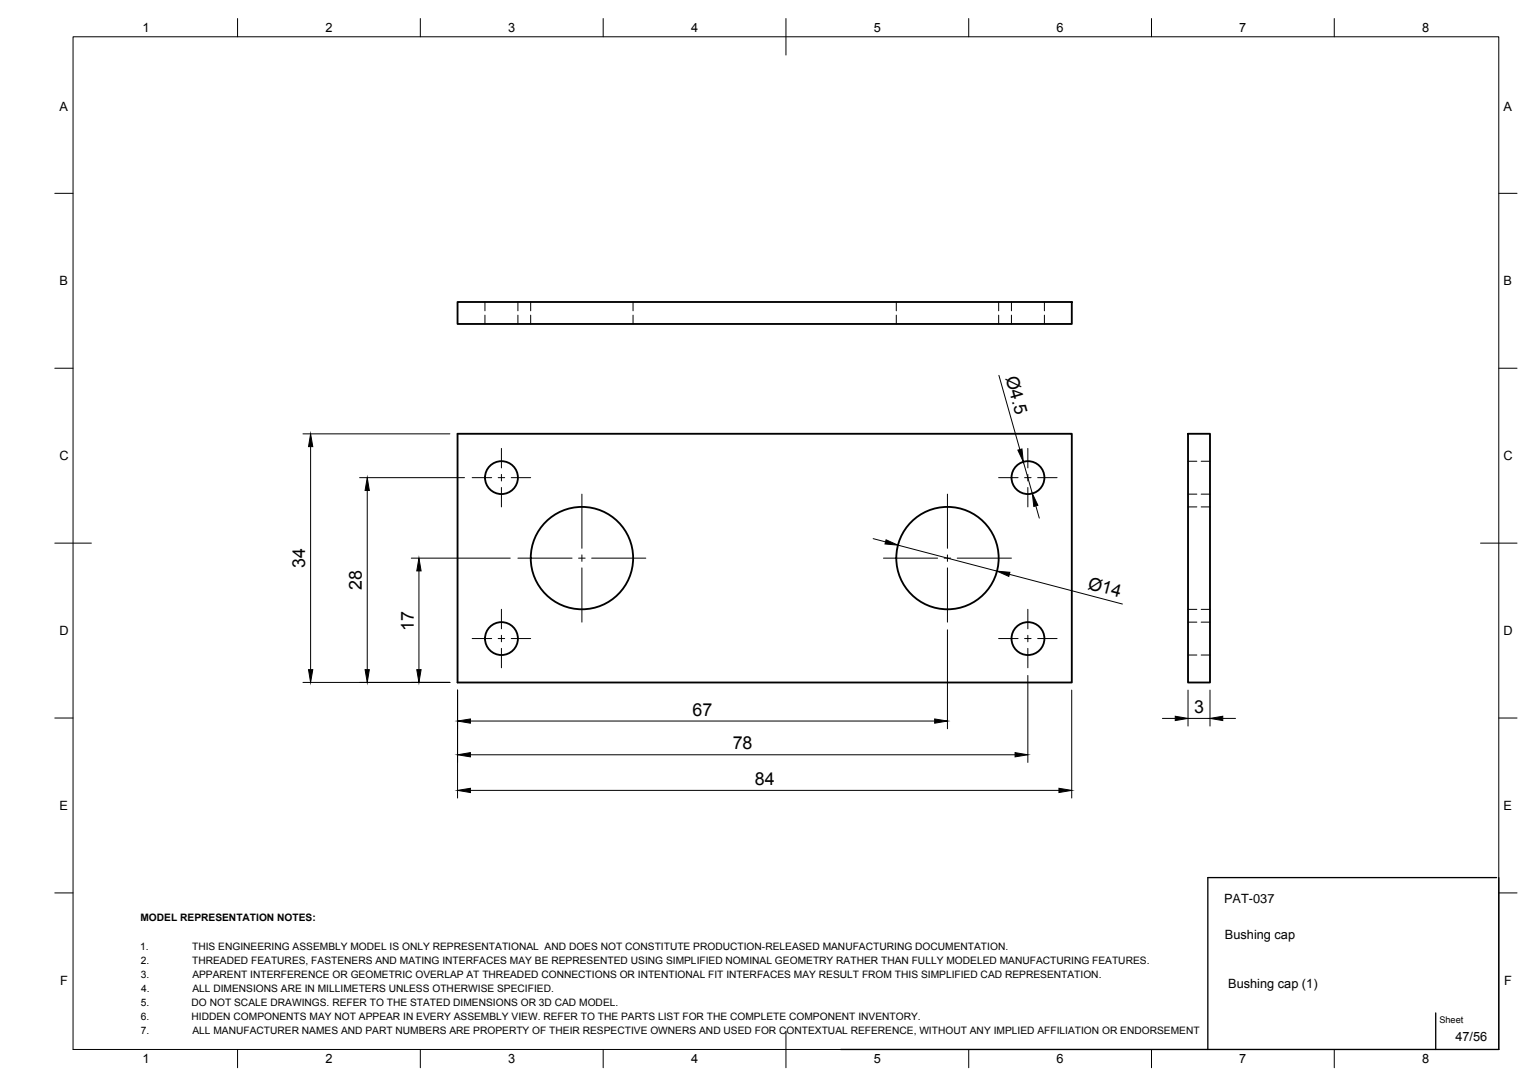
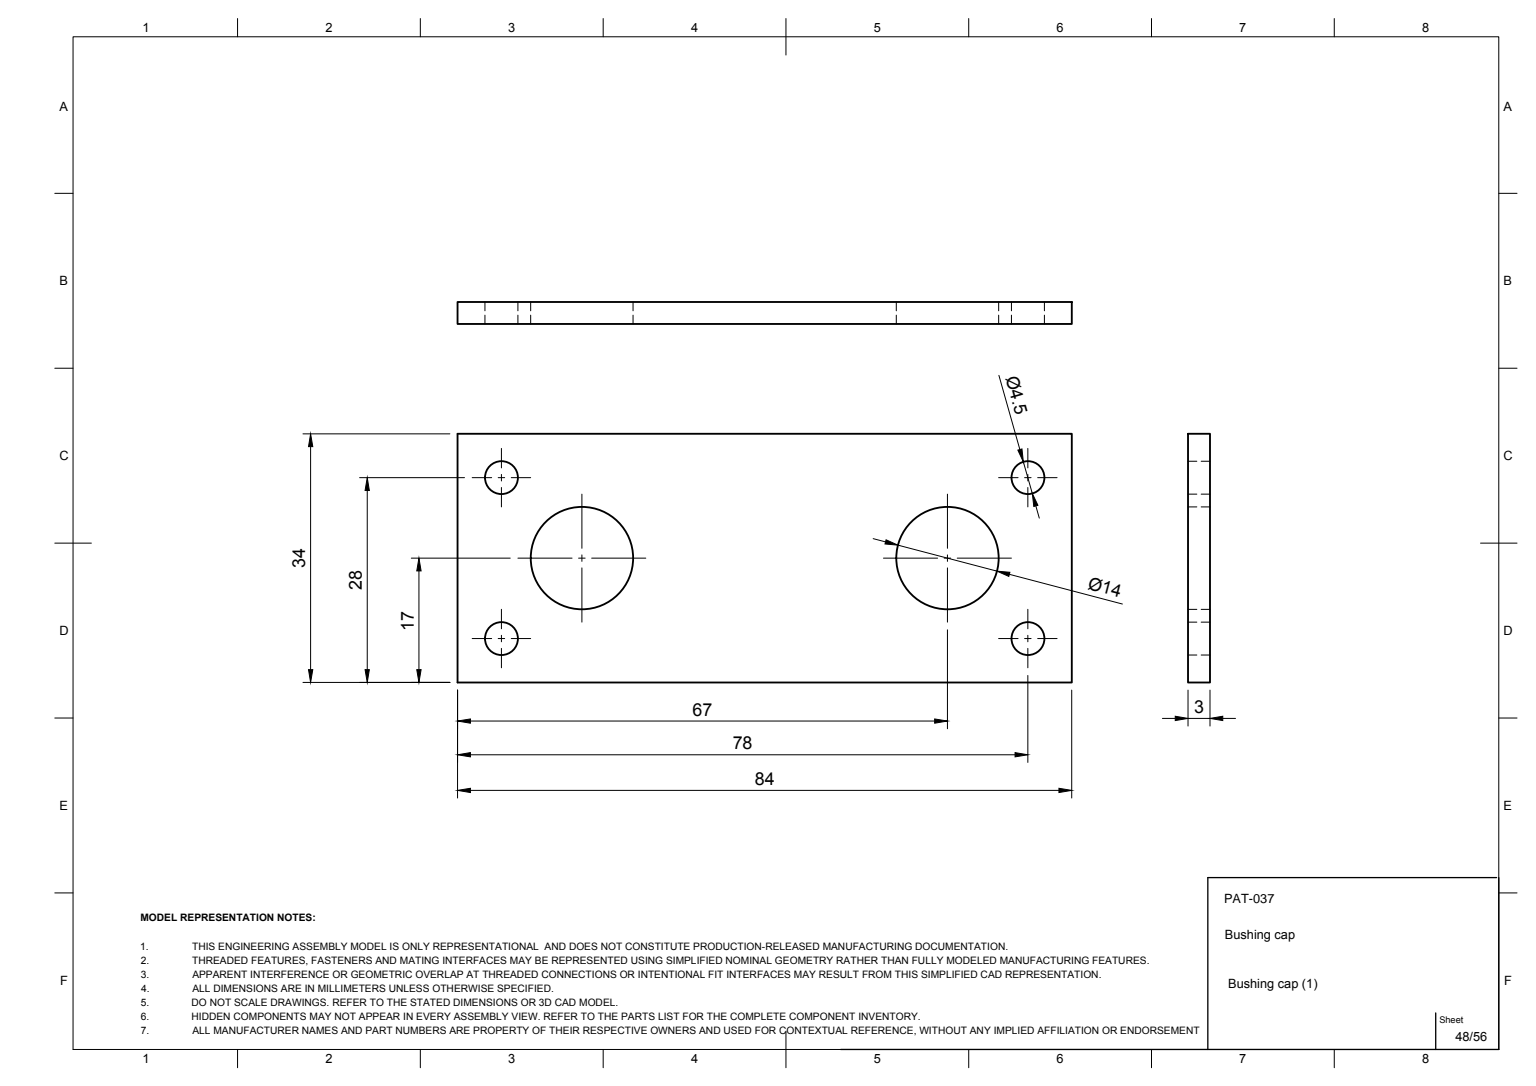
ISO-10303-21;
HEADER;
/* Generated by software containing ST-Developer
 * from STEP Tools, Inc. (www.steptools.com) 
 */

FILE_DESCRIPTION(
/* description */ ('Flywheel Crank-Slider'),
/* implementation_level */ '2;1');

FILE_NAME(
/* name */ 'Bushing cap.step',
/* time_stamp */ '2026-10-28T03:23:13-07:00',
/* author */ (''),
/* organization */ (''),
/* preprocessor_version */ 'ST-DEVELOPER v20.2',
/* originating_system */ 'Autodesk Translation Framework v15.17.0.0',
/* authorisation */ '');

FILE_SCHEMA (('AUTOMOTIVE_DESIGN { 1 0 10303 214 3 1 1 }'));
ENDSEC;

DATA;
#10=MECHANICAL_DESIGN_GEOMETRIC_PRESENTATION_REPRESENTATION('',(#720),#17322);
#607=SHAPE_REPRESENTATION_RELATIONSHIP('SRR','None',#17608,#659);
#659=ADVANCED_BREP_SHAPE_REPRESENTATION('',(#777),#17312);
#720=STYLED_ITEM('',(#17924),#777);
#777=MANIFOLD_SOLID_BREP('Body1',#9102);
#967=FACE_BOUND('',#2496,.T.);
#968=FACE_BOUND('',#2497,.T.);
#969=FACE_BOUND('',#2498,.T.);
#970=FACE_BOUND('',#2499,.T.);
#971=FACE_BOUND('',#2500,.T.);
#972=FACE_BOUND('',#2501,.T.);
#973=FACE_BOUND('',#2504,.T.);
#974=FACE_BOUND('',#2505,.T.);
#975=FACE_BOUND('',#2506,.T.);
#976=FACE_BOUND('',#2507,.T.);
#977=FACE_BOUND('',#2508,.T.);
#978=FACE_BOUND('',#2509,.T.);
#1270=PLANE('',#10587);
#1271=PLANE('',#10588);
#1272=PLANE('',#10589);
#1273=PLANE('',#10590);
#1274=PLANE('',#10591);
#1275=PLANE('',#10592);
#1771=FACE_OUTER_BOUND('',#2488,.T.);
#1772=FACE_OUTER_BOUND('',#2489,.T.);
#1773=FACE_OUTER_BOUND('',#2490,.T.);
#1774=FACE_OUTER_BOUND('',#2491,.T.);
#1775=FACE_OUTER_BOUND('',#2492,.T.);
#1776=FACE_OUTER_BOUND('',#2493,.T.);
#1777=FACE_OUTER_BOUND('',#2494,.T.);
#1778=FACE_OUTER_BOUND('',#2495,.T.);
#1779=FACE_OUTER_BOUND('',#2502,.T.);
#1780=FACE_OUTER_BOUND('',#2503,.T.);
#1781=FACE_OUTER_BOUND('',#2510,.T.);
#1782=FACE_OUTER_BOUND('',#2511,.T.);
#2488=EDGE_LOOP('',(#8000,#8001,#8002,#8003));
#2489=EDGE_LOOP('',(#8004,#8005,#8006,#8007));
#2490=EDGE_LOOP('',(#8008,#8009,#8010,#8011));
#2491=EDGE_LOOP('',(#8012,#8013,#8014,#8015));
#2492=EDGE_LOOP('',(#8016,#8017,#8018,#8019));
#2493=EDGE_LOOP('',(#8020,#8021,#8022,#8023));
#2494=EDGE_LOOP('',(#8024,#8025,#8026,#8027));
#2495=EDGE_LOOP('',(#8028,#8029,#8030,#8031));
#2496=EDGE_LOOP('',(#8032));
#2497=EDGE_LOOP('',(#8033));
#2498=EDGE_LOOP('',(#8034));
#2499=EDGE_LOOP('',(#8035));
#2500=EDGE_LOOP('',(#8036));
#2501=EDGE_LOOP('',(#8037));
#2502=EDGE_LOOP('',(#8038,#8039,#8040,#8041));
#2503=EDGE_LOOP('',(#8042,#8043,#8044,#8045));
#2504=EDGE_LOOP('',(#8046));
#2505=EDGE_LOOP('',(#8047));
#2506=EDGE_LOOP('',(#8048));
#2507=EDGE_LOOP('',(#8049));
#2508=EDGE_LOOP('',(#8050));
#2509=EDGE_LOOP('',(#8051));
#2510=EDGE_LOOP('',(#8052,#8053,#8054,#8055));
#2511=EDGE_LOOP('',(#8056,#8057,#8058,#8059));
#3133=LINE('',#16741,#3744);
#3134=LINE('',#16747,#3745);
#3135=LINE('',#16753,#3746);
#3136=LINE('',#16759,#3747);
#3137=LINE('',#16765,#3748);
#3138=LINE('',#16771,#3749);
#3139=LINE('',#16776,#3750);
#3140=LINE('',#16778,#3751);
#3141=LINE('',#16780,#3752);
#3142=LINE('',#16781,#3753);
#3143=LINE('',#16784,#3754);
#3144=LINE('',#16786,#3755);
#3145=LINE('',#16787,#3756);
#3146=LINE('',#16790,#3757);
#3147=LINE('',#16792,#3758);
#3148=LINE('',#16793,#3759);
#3149=LINE('',#16795,#3760);
#3150=LINE('',#16796,#3761);
#3744=VECTOR('',#13119,0.225);
#3745=VECTOR('',#13126,0.225);
#3746=VECTOR('',#13133,0.225);
#3747=VECTOR('',#13140,0.225);
#3748=VECTOR('',#13147,0.7);
#3749=VECTOR('',#13154,0.7);
#3750=VECTOR('',#13159,1.);
#3751=VECTOR('',#13160,1.);
#3752=VECTOR('',#13161,1.);
#3753=VECTOR('',#13162,1.);
#3754=VECTOR('',#13165,1.);
#3755=VECTOR('',#13166,1.);
#3756=VECTOR('',#13167,1.);
#3757=VECTOR('',#13170,1.);
#3758=VECTOR('',#13171,1.);
#3759=VECTOR('',#13172,1.);
#3760=VECTOR('',#13175,1.);
#3761=VECTOR('',#13176,1.);
#4206=CIRCLE('',#10570,0.225);
#4207=CIRCLE('',#10571,0.225);
#4208=CIRCLE('',#10573,0.225);
#4209=CIRCLE('',#10574,0.225);
#4210=CIRCLE('',#10576,0.225);
#4211=CIRCLE('',#10577,0.225);
#4212=CIRCLE('',#10579,0.225);
#4213=CIRCLE('',#10580,0.225);
#4214=CIRCLE('',#10582,0.7);
#4215=CIRCLE('',#10583,0.7);
#4216=CIRCLE('',#10585,0.7);
#4217=CIRCLE('',#10586,0.7);
#4909=VERTEX_POINT('',#16738);
#4910=VERTEX_POINT('',#16740);
#4911=VERTEX_POINT('',#16744);
#4912=VERTEX_POINT('',#16746);
#4913=VERTEX_POINT('',#16750);
#4914=VERTEX_POINT('',#16752);
#4915=VERTEX_POINT('',#16756);
#4916=VERTEX_POINT('',#16758);
#4917=VERTEX_POINT('',#16762);
#4918=VERTEX_POINT('',#16764);
#4919=VERTEX_POINT('',#16768);
#4920=VERTEX_POINT('',#16770);
#4921=VERTEX_POINT('',#16774);
#4922=VERTEX_POINT('',#16775);
#4923=VERTEX_POINT('',#16777);
#4924=VERTEX_POINT('',#16779);
#4925=VERTEX_POINT('',#16783);
#4926=VERTEX_POINT('',#16785);
#4927=VERTEX_POINT('',#16789);
#4928=VERTEX_POINT('',#16791);
#5957=EDGE_CURVE('',#4909,#4909,#4206,.T.);
#5958=EDGE_CURVE('',#4909,#4910,#3133,.T.);
#5959=EDGE_CURVE('',#4910,#4910,#4207,.T.);
#5960=EDGE_CURVE('',#4911,#4911,#4208,.T.);
#5961=EDGE_CURVE('',#4911,#4912,#3134,.T.);
#5962=EDGE_CURVE('',#4912,#4912,#4209,.T.);
#5963=EDGE_CURVE('',#4913,#4913,#4210,.T.);
#5964=EDGE_CURVE('',#4913,#4914,#3135,.T.);
#5965=EDGE_CURVE('',#4914,#4914,#4211,.T.);
#5966=EDGE_CURVE('',#4915,#4915,#4212,.T.);
#5967=EDGE_CURVE('',#4915,#4916,#3136,.T.);
#5968=EDGE_CURVE('',#4916,#4916,#4213,.T.);
#5969=EDGE_CURVE('',#4917,#4917,#4214,.T.);
#5970=EDGE_CURVE('',#4917,#4918,#3137,.T.);
#5971=EDGE_CURVE('',#4918,#4918,#4215,.T.);
#5972=EDGE_CURVE('',#4919,#4919,#4216,.T.);
#5973=EDGE_CURVE('',#4919,#4920,#3138,.T.);
#5974=EDGE_CURVE('',#4920,#4920,#4217,.T.);
#5975=EDGE_CURVE('',#4921,#4922,#3139,.T.);
#5976=EDGE_CURVE('',#4922,#4923,#3140,.T.);
#5977=EDGE_CURVE('',#4924,#4923,#3141,.T.);
#5978=EDGE_CURVE('',#4921,#4924,#3142,.T.);
#5979=EDGE_CURVE('',#4925,#4921,#3143,.T.);
#5980=EDGE_CURVE('',#4926,#4924,#3144,.T.);
#5981=EDGE_CURVE('',#4925,#4926,#3145,.T.);
#5982=EDGE_CURVE('',#4927,#4925,#3146,.T.);
#5983=EDGE_CURVE('',#4928,#4926,#3147,.T.);
#5984=EDGE_CURVE('',#4927,#4928,#3148,.T.);
#5985=EDGE_CURVE('',#4922,#4927,#3149,.T.);
#5986=EDGE_CURVE('',#4923,#4928,#3150,.T.);
#8000=ORIENTED_EDGE('',*,*,#5957,.F.);
#8001=ORIENTED_EDGE('',*,*,#5958,.T.);
#8002=ORIENTED_EDGE('',*,*,#5959,.F.);
#8003=ORIENTED_EDGE('',*,*,#5958,.F.);
#8004=ORIENTED_EDGE('',*,*,#5960,.F.);
#8005=ORIENTED_EDGE('',*,*,#5961,.T.);
#8006=ORIENTED_EDGE('',*,*,#5962,.F.);
#8007=ORIENTED_EDGE('',*,*,#5961,.F.);
#8008=ORIENTED_EDGE('',*,*,#5963,.F.);
#8009=ORIENTED_EDGE('',*,*,#5964,.T.);
#8010=ORIENTED_EDGE('',*,*,#5965,.F.);
#8011=ORIENTED_EDGE('',*,*,#5964,.F.);
#8012=ORIENTED_EDGE('',*,*,#5966,.F.);
#8013=ORIENTED_EDGE('',*,*,#5967,.T.);
#8014=ORIENTED_EDGE('',*,*,#5968,.F.);
#8015=ORIENTED_EDGE('',*,*,#5967,.F.);
#8016=ORIENTED_EDGE('',*,*,#5969,.F.);
#8017=ORIENTED_EDGE('',*,*,#5970,.T.);
#8018=ORIENTED_EDGE('',*,*,#5971,.F.);
#8019=ORIENTED_EDGE('',*,*,#5970,.F.);
#8020=ORIENTED_EDGE('',*,*,#5972,.F.);
#8021=ORIENTED_EDGE('',*,*,#5973,.T.);
#8022=ORIENTED_EDGE('',*,*,#5974,.F.);
#8023=ORIENTED_EDGE('',*,*,#5973,.F.);
#8024=ORIENTED_EDGE('',*,*,#5975,.T.);
#8025=ORIENTED_EDGE('',*,*,#5976,.T.);
#8026=ORIENTED_EDGE('',*,*,#5977,.F.);
#8027=ORIENTED_EDGE('',*,*,#5978,.F.);
#8028=ORIENTED_EDGE('',*,*,#5979,.T.);
#8029=ORIENTED_EDGE('',*,*,#5978,.T.);
#8030=ORIENTED_EDGE('',*,*,#5980,.F.);
#8031=ORIENTED_EDGE('',*,*,#5981,.F.);
#8032=ORIENTED_EDGE('',*,*,#5974,.T.);
#8033=ORIENTED_EDGE('',*,*,#5971,.T.);
#8034=ORIENTED_EDGE('',*,*,#5968,.T.);
#8035=ORIENTED_EDGE('',*,*,#5965,.T.);
#8036=ORIENTED_EDGE('',*,*,#5962,.T.);
#8037=ORIENTED_EDGE('',*,*,#5959,.T.);
#8038=ORIENTED_EDGE('',*,*,#5982,.T.);
#8039=ORIENTED_EDGE('',*,*,#5981,.T.);
#8040=ORIENTED_EDGE('',*,*,#5983,.F.);
#8041=ORIENTED_EDGE('',*,*,#5984,.F.);
#8042=ORIENTED_EDGE('',*,*,#5985,.T.);
#8043=ORIENTED_EDGE('',*,*,#5984,.T.);
#8044=ORIENTED_EDGE('',*,*,#5986,.F.);
#8045=ORIENTED_EDGE('',*,*,#5976,.F.);
#8046=ORIENTED_EDGE('',*,*,#5972,.T.);
#8047=ORIENTED_EDGE('',*,*,#5969,.T.);
#8048=ORIENTED_EDGE('',*,*,#5966,.T.);
#8049=ORIENTED_EDGE('',*,*,#5963,.T.);
#8050=ORIENTED_EDGE('',*,*,#5960,.T.);
#8051=ORIENTED_EDGE('',*,*,#5957,.T.);
#8052=ORIENTED_EDGE('',*,*,#5986,.T.);
#8053=ORIENTED_EDGE('',*,*,#5983,.T.);
#8054=ORIENTED_EDGE('',*,*,#5980,.T.);
#8055=ORIENTED_EDGE('',*,*,#5977,.T.);
#8056=ORIENTED_EDGE('',*,*,#5985,.F.);
#8057=ORIENTED_EDGE('',*,*,#5975,.F.);
#8058=ORIENTED_EDGE('',*,*,#5979,.F.);
#8059=ORIENTED_EDGE('',*,*,#5982,.F.);
#8480=CYLINDRICAL_SURFACE('',#10569,0.225);
#8481=CYLINDRICAL_SURFACE('',#10572,0.225);
#8482=CYLINDRICAL_SURFACE('',#10575,0.225);
#8483=CYLINDRICAL_SURFACE('',#10578,0.225);
#8484=CYLINDRICAL_SURFACE('',#10581,0.7);
#8485=CYLINDRICAL_SURFACE('',#10584,0.7);
#8962=ADVANCED_FACE('',(#1771),#8480,.F.);
#8963=ADVANCED_FACE('',(#1772),#8481,.F.);
#8964=ADVANCED_FACE('',(#1773),#8482,.F.);
#8965=ADVANCED_FACE('',(#1774),#8483,.F.);
#8966=ADVANCED_FACE('',(#1775),#8484,.F.);
#8967=ADVANCED_FACE('',(#1776),#8485,.F.);
#8968=ADVANCED_FACE('',(#1777),#1270,.T.);
#8969=ADVANCED_FACE('',(#1778,#967,#968,#969,#970,#971,#972),#1271,.T.);
#8970=ADVANCED_FACE('',(#1779),#1272,.T.);
#8971=ADVANCED_FACE('',(#1780,#973,#974,#975,#976,#977,#978),#1273,.T.);
#8972=ADVANCED_FACE('',(#1781),#1274,.T.);
#8973=ADVANCED_FACE('',(#1782),#1275,.F.);
#9102=CLOSED_SHELL('',(#8962,#8963,#8964,#8965,#8966,#8967,#8968,#8969,
#8970,#8971,#8972,#8973));
#10568=AXIS2_PLACEMENT_3D('',#16736,#13113,#13114);
#10569=AXIS2_PLACEMENT_3D('',#16737,#13115,#13116);
#10570=AXIS2_PLACEMENT_3D('',#16739,#13117,#13118);
#10571=AXIS2_PLACEMENT_3D('',#16742,#13120,#13121);
#10572=AXIS2_PLACEMENT_3D('',#16743,#13122,#13123);
#10573=AXIS2_PLACEMENT_3D('',#16745,#13124,#13125);
#10574=AXIS2_PLACEMENT_3D('',#16748,#13127,#13128);
#10575=AXIS2_PLACEMENT_3D('',#16749,#13129,#13130);
#10576=AXIS2_PLACEMENT_3D('',#16751,#13131,#13132);
#10577=AXIS2_PLACEMENT_3D('',#16754,#13134,#13135);
#10578=AXIS2_PLACEMENT_3D('',#16755,#13136,#13137);
#10579=AXIS2_PLACEMENT_3D('',#16757,#13138,#13139);
#10580=AXIS2_PLACEMENT_3D('',#16760,#13141,#13142);
#10581=AXIS2_PLACEMENT_3D('',#16761,#13143,#13144);
#10582=AXIS2_PLACEMENT_3D('',#16763,#13145,#13146);
#10583=AXIS2_PLACEMENT_3D('',#16766,#13148,#13149);
#10584=AXIS2_PLACEMENT_3D('',#16767,#13150,#13151);
#10585=AXIS2_PLACEMENT_3D('',#16769,#13152,#13153);
#10586=AXIS2_PLACEMENT_3D('',#16772,#13155,#13156);
#10587=AXIS2_PLACEMENT_3D('',#16773,#13157,#13158);
#10588=AXIS2_PLACEMENT_3D('',#16782,#13163,#13164);
#10589=AXIS2_PLACEMENT_3D('',#16788,#13168,#13169);
#10590=AXIS2_PLACEMENT_3D('',#16794,#13173,#13174);
#10591=AXIS2_PLACEMENT_3D('',#16797,#13177,#13178);
#10592=AXIS2_PLACEMENT_3D('',#16798,#13179,#13180);
#13113=DIRECTION('axis',(0.,0.,1.));
#13114=DIRECTION('refdir',(1.,0.,0.));
#13115=DIRECTION('center_axis',(1.,0.,0.));
#13116=DIRECTION('ref_axis',(0.,0.,-1.));
#13117=DIRECTION('center_axis',(1.,0.,0.));
#13118=DIRECTION('ref_axis',(0.,0.,-1.));
#13119=DIRECTION('',(1.,0.,0.));
#13120=DIRECTION('center_axis',(-1.,0.,0.));
#13121=DIRECTION('ref_axis',(0.,0.,-1.));
#13122=DIRECTION('center_axis',(1.,0.,0.));
#13123=DIRECTION('ref_axis',(0.,0.,-1.));
#13124=DIRECTION('center_axis',(1.,0.,0.));
#13125=DIRECTION('ref_axis',(0.,0.,-1.));
#13126=DIRECTION('',(1.,0.,0.));
#13127=DIRECTION('center_axis',(-1.,0.,0.));
#13128=DIRECTION('ref_axis',(0.,0.,-1.));
#13129=DIRECTION('center_axis',(1.,0.,0.));
#13130=DIRECTION('ref_axis',(0.,0.,-1.));
#13131=DIRECTION('center_axis',(1.,0.,0.));
#13132=DIRECTION('ref_axis',(0.,0.,-1.));
#13133=DIRECTION('',(1.,0.,0.));
#13134=DIRECTION('center_axis',(-1.,0.,0.));
#13135=DIRECTION('ref_axis',(0.,0.,-1.));
#13136=DIRECTION('center_axis',(1.,0.,0.));
#13137=DIRECTION('ref_axis',(0.,0.,-1.));
#13138=DIRECTION('center_axis',(1.,0.,0.));
#13139=DIRECTION('ref_axis',(0.,0.,-1.));
#13140=DIRECTION('',(1.,0.,0.));
#13141=DIRECTION('center_axis',(-1.,0.,0.));
#13142=DIRECTION('ref_axis',(0.,0.,-1.));
#13143=DIRECTION('center_axis',(1.,0.,0.));
#13144=DIRECTION('ref_axis',(0.,0.,-1.));
#13145=DIRECTION('center_axis',(1.,0.,0.));
#13146=DIRECTION('ref_axis',(0.,0.,-1.));
#13147=DIRECTION('',(1.,0.,0.));
#13148=DIRECTION('center_axis',(-1.,0.,0.));
#13149=DIRECTION('ref_axis',(0.,0.,-1.));
#13150=DIRECTION('center_axis',(1.,0.,0.));
#13151=DIRECTION('ref_axis',(0.,0.,-1.));
#13152=DIRECTION('center_axis',(1.,0.,0.));
#13153=DIRECTION('ref_axis',(0.,0.,-1.));
#13154=DIRECTION('',(1.,0.,0.));
#13155=DIRECTION('center_axis',(-1.,0.,0.));
#13156=DIRECTION('ref_axis',(0.,0.,-1.));
#13157=DIRECTION('center_axis',(0.,1.,0.));
#13158=DIRECTION('ref_axis',(-1.,0.,0.));
#13159=DIRECTION('',(-1.,0.,0.));
#13160=DIRECTION('',(0.,0.,1.));
#13161=DIRECTION('',(-1.,0.,0.));
#13162=DIRECTION('',(0.,0.,1.));
#13163=DIRECTION('center_axis',(1.,0.,0.));
#13164=DIRECTION('ref_axis',(0.,1.,0.));
#13165=DIRECTION('',(0.,1.,0.));
#13166=DIRECTION('',(0.,1.,0.));
#13167=DIRECTION('',(0.,0.,1.));
#13168=DIRECTION('center_axis',(0.,-1.,0.));
#13169=DIRECTION('ref_axis',(1.,0.,0.));
#13170=DIRECTION('',(1.,0.,0.));
#13171=DIRECTION('',(1.,0.,0.));
#13172=DIRECTION('',(0.,0.,1.));
#13173=DIRECTION('center_axis',(-1.,0.,0.));
#13174=DIRECTION('ref_axis',(0.,-1.,0.));
#13175=DIRECTION('',(0.,-1.,0.));
#13176=DIRECTION('',(0.,-1.,0.));
#13177=DIRECTION('center_axis',(0.,0.,1.));
#13178=DIRECTION('ref_axis',(1.,0.,0.));
#13179=DIRECTION('center_axis',(0.,0.,1.));
#13180=DIRECTION('ref_axis',(1.,0.,0.));
#16736=CARTESIAN_POINT('',(0.,0.,0.));
#16737=CARTESIAN_POINT('Origin',(10.,3.6,3.9));
#16738=CARTESIAN_POINT('',(10.1,3.6,4.125));
#16739=CARTESIAN_POINT('Origin',(10.1,3.6,3.9));
#16740=CARTESIAN_POINT('',(10.4,3.6,4.125));
#16741=CARTESIAN_POINT('',(10.,3.6,4.125));
#16742=CARTESIAN_POINT('Origin',(10.4,3.6,3.9));
#16743=CARTESIAN_POINT('Origin',(10.,-3.6,6.1));
#16744=CARTESIAN_POINT('',(10.1,-3.6,6.325));
#16745=CARTESIAN_POINT('Origin',(10.1,-3.6,6.1));
#16746=CARTESIAN_POINT('',(10.4,-3.6,6.325));
#16747=CARTESIAN_POINT('',(10.,-3.6,6.325));
#16748=CARTESIAN_POINT('Origin',(10.4,-3.6,6.1));
#16749=CARTESIAN_POINT('Origin',(10.,-3.6,3.9));
#16750=CARTESIAN_POINT('',(10.1,-3.6,4.125));
#16751=CARTESIAN_POINT('Origin',(10.1,-3.6,3.9));
#16752=CARTESIAN_POINT('',(10.4,-3.6,4.125));
#16753=CARTESIAN_POINT('',(10.,-3.6,4.125));
#16754=CARTESIAN_POINT('Origin',(10.4,-3.6,3.9));
#16755=CARTESIAN_POINT('Origin',(10.,3.6,6.1));
#16756=CARTESIAN_POINT('',(10.1,3.6,6.325));
#16757=CARTESIAN_POINT('Origin',(10.1,3.6,6.1));
#16758=CARTESIAN_POINT('',(10.4,3.6,6.325));
#16759=CARTESIAN_POINT('',(10.,3.6,6.325));
#16760=CARTESIAN_POINT('Origin',(10.4,3.6,6.1));
#16761=CARTESIAN_POINT('Origin',(10.,-2.5,5.));
#16762=CARTESIAN_POINT('',(10.1,-2.5,5.7));
#16763=CARTESIAN_POINT('Origin',(10.1,-2.5,5.));
#16764=CARTESIAN_POINT('',(10.4,-2.5,5.7));
#16765=CARTESIAN_POINT('',(10.,-2.5,5.7));
#16766=CARTESIAN_POINT('Origin',(10.4,-2.5,5.));
#16767=CARTESIAN_POINT('Origin',(10.,2.5,5.));
#16768=CARTESIAN_POINT('',(10.1,2.5,5.7));
#16769=CARTESIAN_POINT('Origin',(10.1,2.5,5.));
#16770=CARTESIAN_POINT('',(10.4,2.5,5.7));
#16771=CARTESIAN_POINT('',(10.,2.5,5.7));
#16772=CARTESIAN_POINT('Origin',(10.4,2.5,5.));
#16773=CARTESIAN_POINT('Origin',(10.4,4.2,3.3));
#16774=CARTESIAN_POINT('',(10.4,4.2,3.3));
#16775=CARTESIAN_POINT('',(10.1,4.2,3.3));
#16776=CARTESIAN_POINT('',(10.4,4.2,3.3));
#16777=CARTESIAN_POINT('',(10.1,4.2,6.7));
#16778=CARTESIAN_POINT('',(10.1,4.2,3.3));
#16779=CARTESIAN_POINT('',(10.4,4.2,6.7));
#16780=CARTESIAN_POINT('',(10.4,4.2,6.7));
#16781=CARTESIAN_POINT('',(10.4,4.2,3.3));
#16782=CARTESIAN_POINT('Origin',(10.4,-4.2,3.3));
#16783=CARTESIAN_POINT('',(10.4,-4.2,3.3));
#16784=CARTESIAN_POINT('',(10.4,-4.2,3.3));
#16785=CARTESIAN_POINT('',(10.4,-4.2,6.7));
#16786=CARTESIAN_POINT('',(10.4,-4.2,6.7));
#16787=CARTESIAN_POINT('',(10.4,-4.2,3.3));
#16788=CARTESIAN_POINT('Origin',(10.1,-4.2,3.3));
#16789=CARTESIAN_POINT('',(10.1,-4.2,3.3));
#16790=CARTESIAN_POINT('',(10.1,-4.2,3.3));
#16791=CARTESIAN_POINT('',(10.1,-4.2,6.7));
#16792=CARTESIAN_POINT('',(10.1,-4.2,6.7));
#16793=CARTESIAN_POINT('',(10.1,-4.2,3.3));
#16794=CARTESIAN_POINT('Origin',(10.1,4.2,3.3));
#16795=CARTESIAN_POINT('',(10.1,4.2,3.3));
#16796=CARTESIAN_POINT('',(10.1,4.2,6.7));
#16797=CARTESIAN_POINT('Origin',(10.25,0.,6.7));
#16798=CARTESIAN_POINT('Origin',(10.25,0.,3.3));
#17251=UNCERTAINTY_MEASURE_WITH_UNIT(LENGTH_MEASURE(0.001),#17323,
'DISTANCE_ACCURACY_VALUE',
'Maximum model space distance between geometric entities at asserted c
onnectivities');
#17261=UNCERTAINTY_MEASURE_WITH_UNIT(LENGTH_MEASURE(0.001),#17323,
'DISTANCE_ACCURACY_VALUE',
'Maximum model space distance between geometric entities at asserted c
onnectivities');
#17312=(
GEOMETRIC_REPRESENTATION_CONTEXT(3)
GLOBAL_UNCERTAINTY_ASSIGNED_CONTEXT((#17251))
GLOBAL_UNIT_ASSIGNED_CONTEXT((#17323,#17325,#17326))
REPRESENTATION_CONTEXT('','3D')
);
#17322=(
GEOMETRIC_REPRESENTATION_CONTEXT(3)
GLOBAL_UNCERTAINTY_ASSIGNED_CONTEXT((#17261))
GLOBAL_UNIT_ASSIGNED_CONTEXT((#17323,#17325,#17326))
REPRESENTATION_CONTEXT('','3D')
);
#17323=(
LENGTH_UNIT()
NAMED_UNIT(*)
SI_UNIT(.CENTI.,.METRE.)
);
#17325=(
NAMED_UNIT(*)
PLANE_ANGLE_UNIT()
SI_UNIT($,.RADIAN.)
);
#17326=(
NAMED_UNIT(*)
SI_UNIT($,.STERADIAN.)
SOLID_ANGLE_UNIT()
);
#17377=SHAPE_DEFINITION_REPRESENTATION(#17451,#17608);
#17451=PRODUCT_DEFINITION_SHAPE('',$,#17669);
#17608=SHAPE_REPRESENTATION('',(#10568),#17312);
#17618=PRODUCT_DEFINITION_CONTEXT('part definition',#17800,'design');
#17669=PRODUCT_DEFINITION('Bushing cap','Bushing cap',#17729,#17618);
#17729=PRODUCT_DEFINITION_FORMATION('',$,#17852);
#17800=APPLICATION_CONTEXT(
'Core Data for Automotive Mechanical Design Process');
#17801=PRODUCT_CONTEXT('part definition',#17800,'mechanical');
#17852=PRODUCT('Bushing cap','Bushing cap','Bushing cap',(#17801));
#17918=COLOUR_RGB('Sky Blue',0.24,0.69,0.87);
#17919=FILL_AREA_STYLE_COLOUR('',#17918);
#17920=FILL_AREA_STYLE('',(#17919));
#17921=SURFACE_STYLE_FILL_AREA(#17920);
#17922=SURFACE_SIDE_STYLE('',(#17921));
#17923=SURFACE_STYLE_USAGE(.BOTH.,#17922);
#17924=PRESENTATION_STYLE_ASSIGNMENT((#17923));
ENDSEC;
END-ISO-10303-21;
